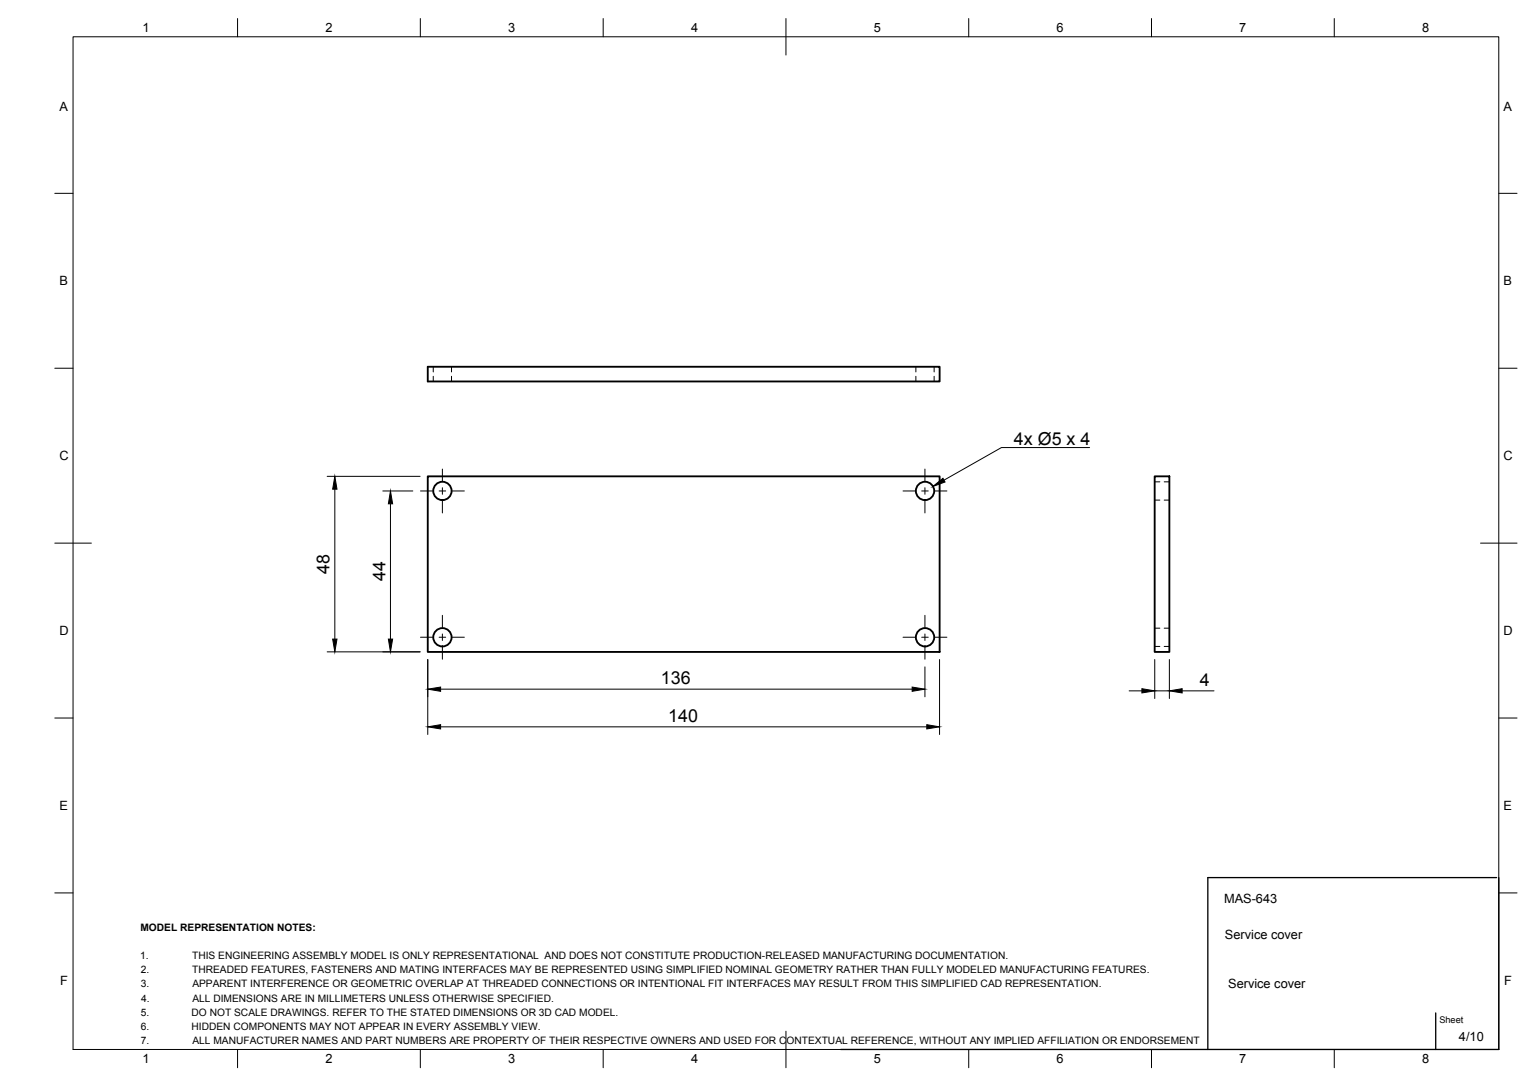
ISO-10303-21;
HEADER;
/* Generated by software containing ST-Developer
 * from STEP Tools, Inc. (www.steptools.com) 
 */

FILE_DESCRIPTION(
/* description */ ('Independent eighteen-tube parallel-flow evaporator geometry. Repeated
 machined headers and gasketed service covers, eighteen copper tubes, 
twenty-nine punched fins, threaded hose connections and bolted mountin
g feet. Native editable features and instanced parts. Braze details, w
orking fluid, pressure and thermal ratings require engineering selecti
on.'),
/* implementation_level */ '2;1');

FILE_NAME(
/* name */ 'Service cover.step',
/* time_stamp */ '2026-11-08T20:53:59-08:00',
/* author */ (''),
/* organization */ (''),
/* preprocessor_version */ 'ST-DEVELOPER v20.2',
/* originating_system */ 'Autodesk Translation Framework v15.17.0.0',
/* authorisation */ '');

FILE_SCHEMA (('AUTOMOTIVE_DESIGN { 1 0 10303 214 3 1 1 }'));
ENDSEC;

DATA;
#10=MECHANICAL_DESIGN_GEOMETRIC_PRESENTATION_REPRESENTATION('',(#334),#42620);
#314=SHAPE_REPRESENTATION_RELATIONSHIP('SRR','None',#42724,#324);
#324=ADVANCED_BREP_SHAPE_REPRESENTATION('',(#344),#42611);
#334=STYLED_ITEM('',(#42783),#344);
#344=MANIFOLD_SOLID_BREP('Body1',#10384);
#401=FACE_BOUND('',#1551,.T.);
#402=FACE_BOUND('',#1552,.T.);
#403=FACE_BOUND('',#1553,.T.);
#404=FACE_BOUND('',#1554,.T.);
#405=FACE_BOUND('',#1556,.T.);
#406=FACE_BOUND('',#1557,.T.);
#407=FACE_BOUND('',#1558,.T.);
#408=FACE_BOUND('',#1559,.T.);
#517=PLANE('',#10934);
#518=PLANE('',#10935);
#519=PLANE('',#10936);
#520=PLANE('',#10937);
#521=PLANE('',#10938);
#522=PLANE('',#10939);
#950=FACE_OUTER_BOUND('',#1542,.T.);
#951=FACE_OUTER_BOUND('',#1543,.T.);
#952=FACE_OUTER_BOUND('',#1544,.T.);
#953=FACE_OUTER_BOUND('',#1545,.T.);
#954=FACE_OUTER_BOUND('',#1546,.T.);
#955=FACE_OUTER_BOUND('',#1547,.T.);
#956=FACE_OUTER_BOUND('',#1548,.T.);
#957=FACE_OUTER_BOUND('',#1549,.T.);
#958=FACE_OUTER_BOUND('',#1550,.T.);
#959=FACE_OUTER_BOUND('',#1555,.T.);
#1542=EDGE_LOOP('',(#8411,#8412,#8413,#8414));
#1543=EDGE_LOOP('',(#8415,#8416,#8417,#8418));
#1544=EDGE_LOOP('',(#8419,#8420,#8421,#8422));
#1545=EDGE_LOOP('',(#8423,#8424,#8425,#8426));
#1546=EDGE_LOOP('',(#8427,#8428,#8429,#8430));
#1547=EDGE_LOOP('',(#8431,#8432,#8433,#8434));
#1548=EDGE_LOOP('',(#8435,#8436,#8437,#8438));
#1549=EDGE_LOOP('',(#8439,#8440,#8441,#8442));
#1550=EDGE_LOOP('',(#8443,#8444,#8445,#8446));
#1551=EDGE_LOOP('',(#8447));
#1552=EDGE_LOOP('',(#8448));
#1553=EDGE_LOOP('',(#8449));
#1554=EDGE_LOOP('',(#8450));
#1555=EDGE_LOOP('',(#8451,#8452,#8453,#8454));
#1556=EDGE_LOOP('',(#8455));
#1557=EDGE_LOOP('',(#8456));
#1558=EDGE_LOOP('',(#8457));
#1559=EDGE_LOOP('',(#8458));
#1911=CIRCLE('',#10923,2.5);
#1912=CIRCLE('',#10924,2.5);
#1913=CIRCLE('',#10926,2.5);
#1914=CIRCLE('',#10927,2.5);
#1915=CIRCLE('',#10929,2.5);
#1916=CIRCLE('',#10930,2.5);
#1917=CIRCLE('',#10932,2.5);
#1918=CIRCLE('',#10933,2.5);
#3118=LINE('',#34843,#3656);
#3119=LINE('',#34849,#3657);
#3120=LINE('',#34855,#3658);
#3121=LINE('',#34861,#3659);
#3122=LINE('',#34866,#3660);
#3123=LINE('',#34868,#3661);
#3124=LINE('',#34870,#3662);
#3125=LINE('',#34871,#3663);
#3126=LINE('',#34874,#3664);
#3127=LINE('',#34876,#3665);
#3128=LINE('',#34877,#3666);
#3129=LINE('',#34880,#3667);
#3130=LINE('',#34882,#3668);
#3131=LINE('',#34883,#3669);
#3132=LINE('',#34885,#3670);
#3133=LINE('',#34886,#3671);
#3656=VECTOR('',#12465,2.5);
#3657=VECTOR('',#12472,2.5);
#3658=VECTOR('',#12479,2.5);
#3659=VECTOR('',#12486,2.5);
#3660=VECTOR('',#12491,10.);
#3661=VECTOR('',#12492,10.);
#3662=VECTOR('',#12493,10.);
#3663=VECTOR('',#12494,10.);
#3664=VECTOR('',#12497,10.);
#3665=VECTOR('',#12498,10.);
#3666=VECTOR('',#12499,10.);
#3667=VECTOR('',#12502,10.);
#3668=VECTOR('',#12503,10.);
#3669=VECTOR('',#12504,10.);
#3670=VECTOR('',#12507,10.);
#3671=VECTOR('',#12508,10.);
#4543=VERTEX_POINT('',#34840);
#4544=VERTEX_POINT('',#34842);
#4545=VERTEX_POINT('',#34846);
#4546=VERTEX_POINT('',#34848);
#4547=VERTEX_POINT('',#34852);
#4548=VERTEX_POINT('',#34854);
#4549=VERTEX_POINT('',#34858);
#4550=VERTEX_POINT('',#34860);
#4551=VERTEX_POINT('',#34864);
#4552=VERTEX_POINT('',#34865);
#4553=VERTEX_POINT('',#34867);
#4554=VERTEX_POINT('',#34869);
#4555=VERTEX_POINT('',#34873);
#4556=VERTEX_POINT('',#34875);
#4557=VERTEX_POINT('',#34879);
#4558=VERTEX_POINT('',#34881);
#5888=EDGE_CURVE('',#4543,#4543,#1911,.T.);
#5889=EDGE_CURVE('',#4543,#4544,#3118,.T.);
#5890=EDGE_CURVE('',#4544,#4544,#1912,.T.);
#5891=EDGE_CURVE('',#4545,#4545,#1913,.T.);
#5892=EDGE_CURVE('',#4545,#4546,#3119,.T.);
#5893=EDGE_CURVE('',#4546,#4546,#1914,.T.);
#5894=EDGE_CURVE('',#4547,#4547,#1915,.T.);
#5895=EDGE_CURVE('',#4547,#4548,#3120,.T.);
#5896=EDGE_CURVE('',#4548,#4548,#1916,.T.);
#5897=EDGE_CURVE('',#4549,#4549,#1917,.T.);
#5898=EDGE_CURVE('',#4549,#4550,#3121,.T.);
#5899=EDGE_CURVE('',#4550,#4550,#1918,.T.);
#5900=EDGE_CURVE('',#4551,#4552,#3122,.T.);
#5901=EDGE_CURVE('',#4552,#4553,#3123,.T.);
#5902=EDGE_CURVE('',#4554,#4553,#3124,.T.);
#5903=EDGE_CURVE('',#4551,#4554,#3125,.T.);
#5904=EDGE_CURVE('',#4555,#4551,#3126,.T.);
#5905=EDGE_CURVE('',#4556,#4554,#3127,.T.);
#5906=EDGE_CURVE('',#4555,#4556,#3128,.T.);
#5907=EDGE_CURVE('',#4557,#4555,#3129,.T.);
#5908=EDGE_CURVE('',#4558,#4556,#3130,.T.);
#5909=EDGE_CURVE('',#4557,#4558,#3131,.T.);
#5910=EDGE_CURVE('',#4552,#4557,#3132,.T.);
#5911=EDGE_CURVE('',#4553,#4558,#3133,.T.);
#8411=ORIENTED_EDGE('',*,*,#5888,.F.);
#8412=ORIENTED_EDGE('',*,*,#5889,.T.);
#8413=ORIENTED_EDGE('',*,*,#5890,.F.);
#8414=ORIENTED_EDGE('',*,*,#5889,.F.);
#8415=ORIENTED_EDGE('',*,*,#5891,.F.);
#8416=ORIENTED_EDGE('',*,*,#5892,.T.);
#8417=ORIENTED_EDGE('',*,*,#5893,.F.);
#8418=ORIENTED_EDGE('',*,*,#5892,.F.);
#8419=ORIENTED_EDGE('',*,*,#5894,.F.);
#8420=ORIENTED_EDGE('',*,*,#5895,.T.);
#8421=ORIENTED_EDGE('',*,*,#5896,.F.);
#8422=ORIENTED_EDGE('',*,*,#5895,.F.);
#8423=ORIENTED_EDGE('',*,*,#5897,.F.);
#8424=ORIENTED_EDGE('',*,*,#5898,.T.);
#8425=ORIENTED_EDGE('',*,*,#5899,.F.);
#8426=ORIENTED_EDGE('',*,*,#5898,.F.);
#8427=ORIENTED_EDGE('',*,*,#5900,.T.);
#8428=ORIENTED_EDGE('',*,*,#5901,.T.);
#8429=ORIENTED_EDGE('',*,*,#5902,.F.);
#8430=ORIENTED_EDGE('',*,*,#5903,.F.);
#8431=ORIENTED_EDGE('',*,*,#5904,.T.);
#8432=ORIENTED_EDGE('',*,*,#5903,.T.);
#8433=ORIENTED_EDGE('',*,*,#5905,.F.);
#8434=ORIENTED_EDGE('',*,*,#5906,.F.);
#8435=ORIENTED_EDGE('',*,*,#5907,.T.);
#8436=ORIENTED_EDGE('',*,*,#5906,.T.);
#8437=ORIENTED_EDGE('',*,*,#5908,.F.);
#8438=ORIENTED_EDGE('',*,*,#5909,.F.);
#8439=ORIENTED_EDGE('',*,*,#5910,.T.);
#8440=ORIENTED_EDGE('',*,*,#5909,.T.);
#8441=ORIENTED_EDGE('',*,*,#5911,.F.);
#8442=ORIENTED_EDGE('',*,*,#5901,.F.);
#8443=ORIENTED_EDGE('',*,*,#5911,.T.);
#8444=ORIENTED_EDGE('',*,*,#5908,.T.);
#8445=ORIENTED_EDGE('',*,*,#5905,.T.);
#8446=ORIENTED_EDGE('',*,*,#5902,.T.);
#8447=ORIENTED_EDGE('',*,*,#5888,.T.);
#8448=ORIENTED_EDGE('',*,*,#5891,.T.);
#8449=ORIENTED_EDGE('',*,*,#5894,.T.);
#8450=ORIENTED_EDGE('',*,*,#5897,.T.);
#8451=ORIENTED_EDGE('',*,*,#5910,.F.);
#8452=ORIENTED_EDGE('',*,*,#5900,.F.);
#8453=ORIENTED_EDGE('',*,*,#5904,.F.);
#8454=ORIENTED_EDGE('',*,*,#5907,.F.);
#8455=ORIENTED_EDGE('',*,*,#5890,.T.);
#8456=ORIENTED_EDGE('',*,*,#5893,.T.);
#8457=ORIENTED_EDGE('',*,*,#5896,.T.);
#8458=ORIENTED_EDGE('',*,*,#5899,.T.);
#9712=CYLINDRICAL_SURFACE('',#10922,2.5);
#9713=CYLINDRICAL_SURFACE('',#10925,2.5);
#9714=CYLINDRICAL_SURFACE('',#10928,2.5);
#9715=CYLINDRICAL_SURFACE('',#10931,2.5);
#10186=ADVANCED_FACE('',(#950),#9712,.F.);
#10187=ADVANCED_FACE('',(#951),#9713,.F.);
#10188=ADVANCED_FACE('',(#952),#9714,.F.);
#10189=ADVANCED_FACE('',(#953),#9715,.F.);
#10190=ADVANCED_FACE('',(#954),#517,.T.);
#10191=ADVANCED_FACE('',(#955),#518,.T.);
#10192=ADVANCED_FACE('',(#956),#519,.T.);
#10193=ADVANCED_FACE('',(#957),#520,.T.);
#10194=ADVANCED_FACE('',(#958,#401,#402,#403,#404),#521,.T.);
#10195=ADVANCED_FACE('',(#959,#405,#406,#407,#408),#522,.F.);
#10384=CLOSED_SHELL('',(#10186,#10187,#10188,#10189,#10190,#10191,#10192,
#10193,#10194,#10195));
#10921=AXIS2_PLACEMENT_3D('',#34838,#12459,#12460);
#10922=AXIS2_PLACEMENT_3D('',#34839,#12461,#12462);
#10923=AXIS2_PLACEMENT_3D('',#34841,#12463,#12464);
#10924=AXIS2_PLACEMENT_3D('',#34844,#12466,#12467);
#10925=AXIS2_PLACEMENT_3D('',#34845,#12468,#12469);
#10926=AXIS2_PLACEMENT_3D('',#34847,#12470,#12471);
#10927=AXIS2_PLACEMENT_3D('',#34850,#12473,#12474);
#10928=AXIS2_PLACEMENT_3D('',#34851,#12475,#12476);
#10929=AXIS2_PLACEMENT_3D('',#34853,#12477,#12478);
#10930=AXIS2_PLACEMENT_3D('',#34856,#12480,#12481);
#10931=AXIS2_PLACEMENT_3D('',#34857,#12482,#12483);
#10932=AXIS2_PLACEMENT_3D('',#34859,#12484,#12485);
#10933=AXIS2_PLACEMENT_3D('',#34862,#12487,#12488);
#10934=AXIS2_PLACEMENT_3D('',#34863,#12489,#12490);
#10935=AXIS2_PLACEMENT_3D('',#34872,#12495,#12496);
#10936=AXIS2_PLACEMENT_3D('',#34878,#12500,#12501);
#10937=AXIS2_PLACEMENT_3D('',#34884,#12505,#12506);
#10938=AXIS2_PLACEMENT_3D('',#34887,#12509,#12510);
#10939=AXIS2_PLACEMENT_3D('',#34888,#12511,#12512);
#12459=DIRECTION('axis',(0.,0.,1.));
#12460=DIRECTION('refdir',(1.,0.,0.));
#12461=DIRECTION('center_axis',(0.,0.,-1.));
#12462=DIRECTION('ref_axis',(1.,0.,0.));
#12463=DIRECTION('center_axis',(0.,0.,-1.));
#12464=DIRECTION('ref_axis',(1.,0.,0.));
#12465=DIRECTION('',(0.,0.,-1.));
#12466=DIRECTION('center_axis',(0.,0.,1.));
#12467=DIRECTION('ref_axis',(1.,0.,0.));
#12468=DIRECTION('center_axis',(0.,0.,-1.));
#12469=DIRECTION('ref_axis',(1.,0.,0.));
#12470=DIRECTION('center_axis',(0.,0.,-1.));
#12471=DIRECTION('ref_axis',(1.,0.,0.));
#12472=DIRECTION('',(0.,0.,-1.));
#12473=DIRECTION('center_axis',(0.,0.,1.));
#12474=DIRECTION('ref_axis',(1.,0.,0.));
#12475=DIRECTION('center_axis',(0.,0.,-1.));
#12476=DIRECTION('ref_axis',(1.,0.,0.));
#12477=DIRECTION('center_axis',(0.,0.,-1.));
#12478=DIRECTION('ref_axis',(1.,0.,0.));
#12479=DIRECTION('',(0.,0.,-1.));
#12480=DIRECTION('center_axis',(0.,0.,1.));
#12481=DIRECTION('ref_axis',(1.,0.,0.));
#12482=DIRECTION('center_axis',(0.,0.,-1.));
#12483=DIRECTION('ref_axis',(1.,0.,0.));
#12484=DIRECTION('center_axis',(0.,0.,-1.));
#12485=DIRECTION('ref_axis',(1.,0.,0.));
#12486=DIRECTION('',(0.,0.,-1.));
#12487=DIRECTION('center_axis',(0.,0.,1.));
#12488=DIRECTION('ref_axis',(1.,0.,0.));
#12489=DIRECTION('center_axis',(0.,1.,0.));
#12490=DIRECTION('ref_axis',(-1.,0.,0.));
#12491=DIRECTION('',(-1.,0.,0.));
#12492=DIRECTION('',(0.,0.,1.));
#12493=DIRECTION('',(-1.,0.,0.));
#12494=DIRECTION('',(0.,0.,1.));
#12495=DIRECTION('center_axis',(1.,0.,0.));
#12496=DIRECTION('ref_axis',(0.,1.,0.));
#12497=DIRECTION('',(0.,1.,0.));
#12498=DIRECTION('',(0.,1.,0.));
#12499=DIRECTION('',(0.,0.,1.));
#12500=DIRECTION('center_axis',(0.,-1.,0.));
#12501=DIRECTION('ref_axis',(1.,0.,0.));
#12502=DIRECTION('',(1.,0.,0.));
#12503=DIRECTION('',(1.,0.,0.));
#12504=DIRECTION('',(0.,0.,1.));
#12505=DIRECTION('center_axis',(-1.,0.,0.));
#12506=DIRECTION('ref_axis',(0.,-1.,0.));
#12507=DIRECTION('',(0.,-1.,0.));
#12508=DIRECTION('',(0.,-1.,0.));
#12509=DIRECTION('center_axis',(0.,0.,1.));
#12510=DIRECTION('ref_axis',(1.,0.,0.));
#12511=DIRECTION('center_axis',(0.,0.,1.));
#12512=DIRECTION('ref_axis',(1.,0.,0.));
#34838=CARTESIAN_POINT('',(0.,0.,0.));
#34839=CARTESIAN_POINT('Origin',(20.,-66.,39.));
#34840=CARTESIAN_POINT('',(17.5,-66.,41.));
#34841=CARTESIAN_POINT('Origin',(20.,-66.,41.));
#34842=CARTESIAN_POINT('',(17.5,-66.,37.));
#34843=CARTESIAN_POINT('',(17.5,-66.,39.));
#34844=CARTESIAN_POINT('Origin',(20.,-66.,37.));
#34845=CARTESIAN_POINT('Origin',(-20.,-66.,39.));
#34846=CARTESIAN_POINT('',(-22.5,-66.,41.));
#34847=CARTESIAN_POINT('Origin',(-20.,-66.,41.));
#34848=CARTESIAN_POINT('',(-22.5,-66.,37.));
#34849=CARTESIAN_POINT('',(-22.5,-66.,39.));
#34850=CARTESIAN_POINT('Origin',(-20.,-66.,37.));
#34851=CARTESIAN_POINT('Origin',(-20.,66.,39.));
#34852=CARTESIAN_POINT('',(-22.5,66.,41.));
#34853=CARTESIAN_POINT('Origin',(-20.,66.,41.));
#34854=CARTESIAN_POINT('',(-22.5,66.,37.));
#34855=CARTESIAN_POINT('',(-22.5,66.,39.));
#34856=CARTESIAN_POINT('Origin',(-20.,66.,37.));
#34857=CARTESIAN_POINT('Origin',(20.,66.,39.));
#34858=CARTESIAN_POINT('',(17.5,66.,41.));
#34859=CARTESIAN_POINT('Origin',(20.,66.,41.));
#34860=CARTESIAN_POINT('',(17.5,66.,37.));
#34861=CARTESIAN_POINT('',(17.5,66.,39.));
#34862=CARTESIAN_POINT('Origin',(20.,66.,37.));
#34863=CARTESIAN_POINT('Origin',(24.,70.,37.));
#34864=CARTESIAN_POINT('',(24.,70.,37.));
#34865=CARTESIAN_POINT('',(-24.,70.,37.));
#34866=CARTESIAN_POINT('',(24.,70.,37.));
#34867=CARTESIAN_POINT('',(-24.,70.,41.));
#34868=CARTESIAN_POINT('',(-24.,70.,37.));
#34869=CARTESIAN_POINT('',(24.,70.,41.));
#34870=CARTESIAN_POINT('',(24.,70.,41.));
#34871=CARTESIAN_POINT('',(24.,70.,37.));
#34872=CARTESIAN_POINT('Origin',(24.,-70.,37.));
#34873=CARTESIAN_POINT('',(24.,-70.,37.));
#34874=CARTESIAN_POINT('',(24.,-70.,37.));
#34875=CARTESIAN_POINT('',(24.,-70.,41.));
#34876=CARTESIAN_POINT('',(24.,-70.,41.));
#34877=CARTESIAN_POINT('',(24.,-70.,37.));
#34878=CARTESIAN_POINT('Origin',(-24.,-70.,37.));
#34879=CARTESIAN_POINT('',(-24.,-70.,37.));
#34880=CARTESIAN_POINT('',(-24.,-70.,37.));
#34881=CARTESIAN_POINT('',(-24.,-70.,41.));
#34882=CARTESIAN_POINT('',(-24.,-70.,41.));
#34883=CARTESIAN_POINT('',(-24.,-70.,37.));
#34884=CARTESIAN_POINT('Origin',(-24.,70.,37.));
#34885=CARTESIAN_POINT('',(-24.,70.,37.));
#34886=CARTESIAN_POINT('',(-24.,70.,41.));
#34887=CARTESIAN_POINT('Origin',(0.,0.,41.));
#34888=CARTESIAN_POINT('Origin',(0.,0.,37.));
#42599=UNCERTAINTY_MEASURE_WITH_UNIT(LENGTH_MEASURE(0.01),#42621,
'DISTANCE_ACCURACY_VALUE',
'Maximum model space distance between geometric entities at asserted c
onnectivities');
#42608=UNCERTAINTY_MEASURE_WITH_UNIT(LENGTH_MEASURE(0.01),#42621,
'DISTANCE_ACCURACY_VALUE',
'Maximum model space distance between geometric entities at asserted c
onnectivities');
#42611=(
GEOMETRIC_REPRESENTATION_CONTEXT(3)
GLOBAL_UNCERTAINTY_ASSIGNED_CONTEXT((#42599))
GLOBAL_UNIT_ASSIGNED_CONTEXT((#42621,#42623,#42624))
REPRESENTATION_CONTEXT('','3D')
);
#42620=(
GEOMETRIC_REPRESENTATION_CONTEXT(3)
GLOBAL_UNCERTAINTY_ASSIGNED_CONTEXT((#42608))
GLOBAL_UNIT_ASSIGNED_CONTEXT((#42621,#42623,#42624))
REPRESENTATION_CONTEXT('','3D')
);
#42621=(
LENGTH_UNIT()
NAMED_UNIT(*)
SI_UNIT(.MILLI.,.METRE.)
);
#42623=(
NAMED_UNIT(*)
PLANE_ANGLE_UNIT()
SI_UNIT($,.RADIAN.)
);
#42624=(
NAMED_UNIT(*)
SI_UNIT($,.STERADIAN.)
SOLID_ANGLE_UNIT()
);
#42627=SHAPE_DEFINITION_REPRESENTATION(#42638,#42724);
#42638=PRODUCT_DEFINITION_SHAPE('',$,#42736);
#42724=SHAPE_REPRESENTATION('',(#10921),#42611);
#42733=PRODUCT_DEFINITION_CONTEXT('part definition',#42768,'design');
#42736=PRODUCT_DEFINITION('Service cover','Service cover',#42747,#42733);
#42747=PRODUCT_DEFINITION_FORMATION('',$,#42772);
#42768=APPLICATION_CONTEXT(
'Core Data for Automotive Mechanical Design Process');
#42769=PRODUCT_CONTEXT('part definition',#42768,'mechanical');
#42772=PRODUCT('Service cover','Service cover',$,(#42769));
#42783=PRESENTATION_STYLE_ASSIGNMENT((#42791));
#42791=SURFACE_STYLE_USAGE(.BOTH.,#42799);
#42799=SURFACE_SIDE_STYLE('',(#42807));
#42807=SURFACE_STYLE_FILL_AREA(#42815);
#42815=FILL_AREA_STYLE('Sky blue',(#42823));
#42823=FILL_AREA_STYLE_COLOUR('Sky blue',#42831);
#42831=COLOUR_RGB('Sky blue',0.317647058823529,0.686274509803922,0.890196078431372);
ENDSEC;
END-ISO-10303-21;
